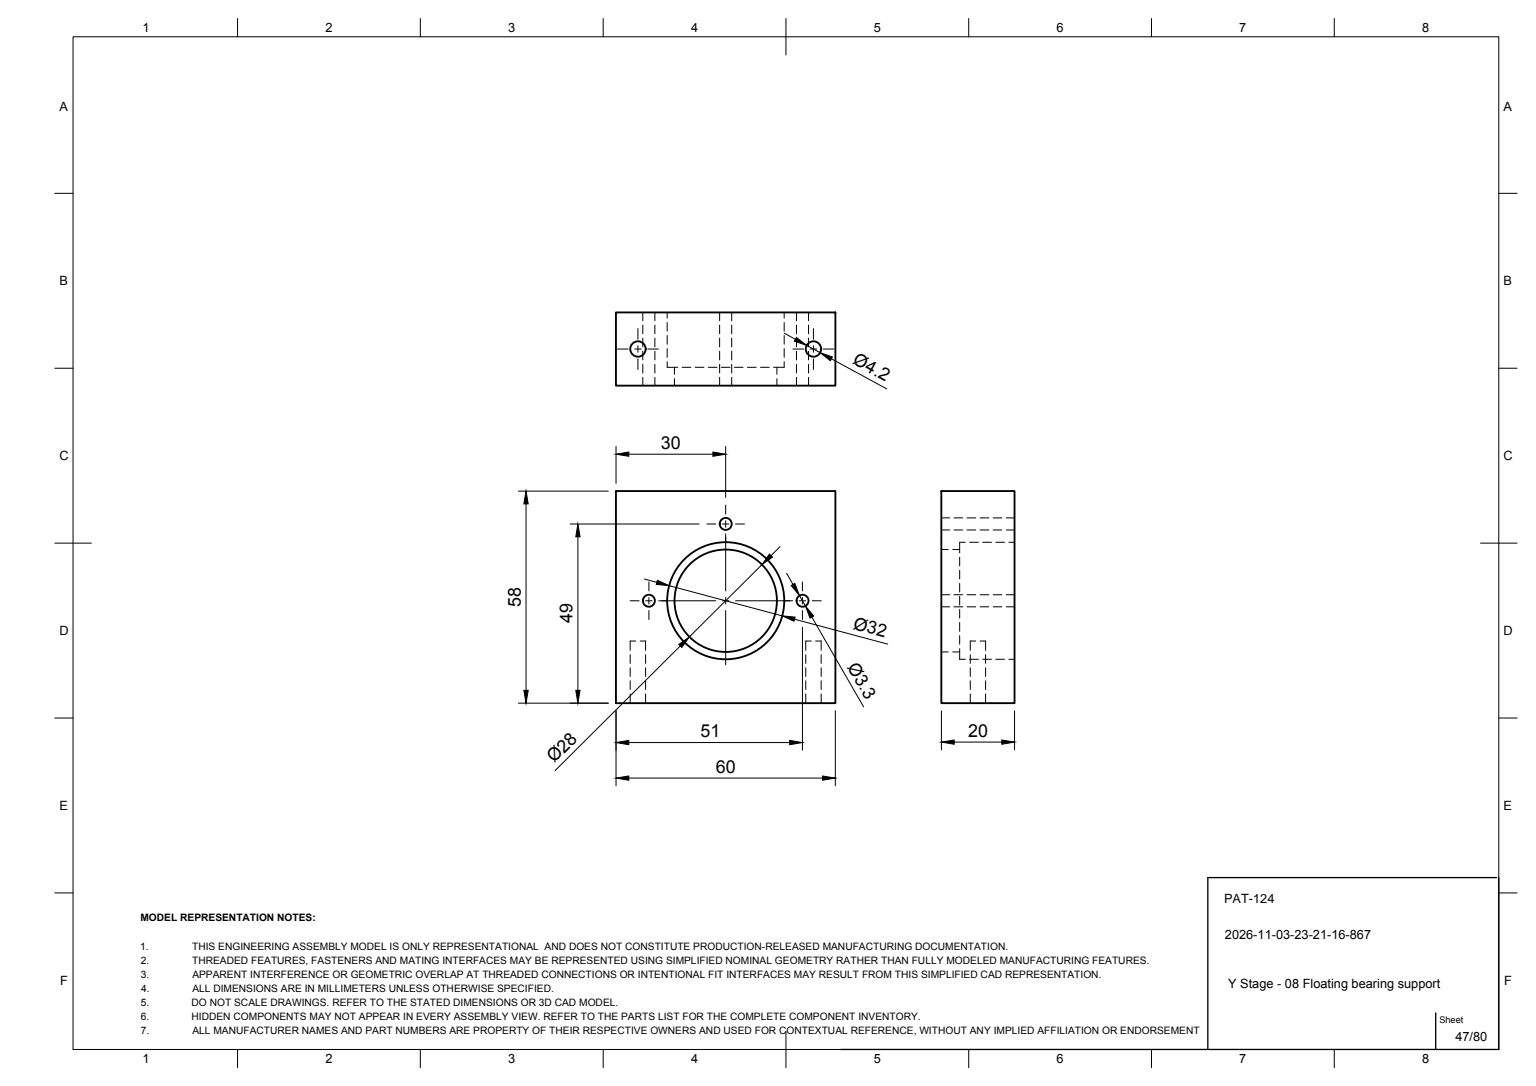
ISO-10303-21;
HEADER;
/* Generated by software containing ST-Developer
 * from STEP Tools, Inc. (www.steptools.com) 
 */

FILE_DESCRIPTION(
/* description */ ('XY cross-slide table'),
/* implementation_level */ '2;1');

FILE_NAME(
/* name */ 'Y Stage - 08 Floating bearing support.step',
/* time_stamp */ '2026-10-28T03:22:46-07:00',
/* author */ (''),
/* organization */ (''),
/* preprocessor_version */ 'ST-DEVELOPER v20.2',
/* originating_system */ 'Autodesk Translation Framework v15.17.0.0',
/* authorisation */ '');

FILE_SCHEMA (('AUTOMOTIVE_DESIGN { 1 0 10303 214 3 1 1 }'));
ENDSEC;

DATA;
#10=MECHANICAL_DESIGN_GEOMETRIC_PRESENTATION_REPRESENTATION('',(#1729),#62984);
#1548=SHAPE_REPRESENTATION_RELATIONSHIP('SRR','None',#63403,#1631);
#1631=ADVANCED_BREP_SHAPE_REPRESENTATION('',(#1838),#62940);
#1729=STYLED_ITEM('',(#63912),#1838);
#1838=MANIFOLD_SOLID_BREP('Body1',#23027);
#2143=FACE_BOUND('',#5155,.T.);
#2144=FACE_BOUND('',#5163,.T.);
#2145=FACE_BOUND('',#5164,.T.);
#2146=FACE_BOUND('',#5165,.T.);
#2147=FACE_BOUND('',#5166,.T.);
#2148=FACE_BOUND('',#5169,.T.);
#2149=FACE_BOUND('',#5170,.T.);
#2150=FACE_BOUND('',#5171,.T.);
#2151=FACE_BOUND('',#5172,.T.);
#2152=FACE_BOUND('',#5175,.T.);
#2153=FACE_BOUND('',#5176,.T.);
#2605=PLANE('',#25365);
#2606=PLANE('',#25372);
#2607=PLANE('',#25376);
#2608=PLANE('',#25377);
#2609=PLANE('',#25378);
#2610=PLANE('',#25379);
#2611=PLANE('',#25380);
#2612=PLANE('',#25381);
#2613=PLANE('',#25382);
#3580=FACE_OUTER_BOUND('',#5150,.T.);
#3581=FACE_OUTER_BOUND('',#5151,.T.);
#3582=FACE_OUTER_BOUND('',#5152,.T.);
#3583=FACE_OUTER_BOUND('',#5153,.T.);
#3584=FACE_OUTER_BOUND('',#5154,.T.);
#3585=FACE_OUTER_BOUND('',#5156,.T.);
#3586=FACE_OUTER_BOUND('',#5157,.T.);
#3587=FACE_OUTER_BOUND('',#5158,.T.);
#3588=FACE_OUTER_BOUND('',#5159,.T.);
#3589=FACE_OUTER_BOUND('',#5160,.T.);
#3590=FACE_OUTER_BOUND('',#5161,.T.);
#3591=FACE_OUTER_BOUND('',#5162,.T.);
#3592=FACE_OUTER_BOUND('',#5167,.T.);
#3593=FACE_OUTER_BOUND('',#5168,.T.);
#3594=FACE_OUTER_BOUND('',#5173,.T.);
#3595=FACE_OUTER_BOUND('',#5174,.T.);
#5150=EDGE_LOOP('',(#18226,#18227,#18228,#18229));
#5151=EDGE_LOOP('',(#18230,#18231,#18232,#18233));
#5152=EDGE_LOOP('',(#18234,#18235,#18236,#18237));
#5153=EDGE_LOOP('',(#18238,#18239,#18240,#18241));
#5154=EDGE_LOOP('',(#18242));
#5155=EDGE_LOOP('',(#18243));
#5156=EDGE_LOOP('',(#18244,#18245,#18246,#18247));
#5157=EDGE_LOOP('',(#18248,#18249,#18250,#18251));
#5158=EDGE_LOOP('',(#18252));
#5159=EDGE_LOOP('',(#18253,#18254,#18255,#18256));
#5160=EDGE_LOOP('',(#18257));
#5161=EDGE_LOOP('',(#18258,#18259,#18260,#18261));
#5162=EDGE_LOOP('',(#18262,#18263,#18264,#18265));
#5163=EDGE_LOOP('',(#18266));
#5164=EDGE_LOOP('',(#18267));
#5165=EDGE_LOOP('',(#18268));
#5166=EDGE_LOOP('',(#18269));
#5167=EDGE_LOOP('',(#18270,#18271,#18272,#18273));
#5168=EDGE_LOOP('',(#18274,#18275,#18276,#18277));
#5169=EDGE_LOOP('',(#18278));
#5170=EDGE_LOOP('',(#18279));
#5171=EDGE_LOOP('',(#18280));
#5172=EDGE_LOOP('',(#18281));
#5173=EDGE_LOOP('',(#18282,#18283,#18284,#18285));
#5174=EDGE_LOOP('',(#18286,#18287,#18288,#18289));
#5175=EDGE_LOOP('',(#18290));
#5176=EDGE_LOOP('',(#18291));
#6712=LINE('',#48100,#8199);
#6713=LINE('',#48106,#8200);
#6714=LINE('',#48112,#8201);
#6715=LINE('',#48118,#8202);
#6716=LINE('',#48125,#8203);
#6717=LINE('',#48131,#8204);
#6718=LINE('',#48138,#8205);
#6719=LINE('',#48144,#8206);
#6720=LINE('',#48146,#8207);
#6721=LINE('',#48148,#8208);
#6722=LINE('',#48149,#8209);
#6723=LINE('',#48152,#8210);
#6724=LINE('',#48154,#8211);
#6725=LINE('',#48155,#8212);
#6726=LINE('',#48158,#8213);
#6727=LINE('',#48160,#8214);
#6728=LINE('',#48161,#8215);
#6729=LINE('',#48163,#8216);
#6730=LINE('',#48164,#8217);
#8199=VECTOR('',#29977,0.165);
#8200=VECTOR('',#29984,0.165);
#8201=VECTOR('',#29991,0.165);
#8202=VECTOR('',#29998,1.6);
#8203=VECTOR('',#30007,1.4);
#8204=VECTOR('',#30014,0.21);
#8205=VECTOR('',#30023,0.21);
#8206=VECTOR('',#30030,1.);
#8207=VECTOR('',#30031,1.);
#8208=VECTOR('',#30032,1.);
#8209=VECTOR('',#30033,1.);
#8210=VECTOR('',#30036,1.);
#8211=VECTOR('',#30037,1.);
#8212=VECTOR('',#30038,1.);
#8213=VECTOR('',#30041,1.);
#8214=VECTOR('',#30042,1.);
#8215=VECTOR('',#30043,1.);
#8216=VECTOR('',#30046,1.);
#8217=VECTOR('',#30047,1.);
#9391=CIRCLE('',#25354,0.165);
#9392=CIRCLE('',#25355,0.165);
#9393=CIRCLE('',#25357,0.165);
#9394=CIRCLE('',#25358,0.165);
#9395=CIRCLE('',#25360,0.165);
#9396=CIRCLE('',#25361,0.165);
#9397=CIRCLE('',#25363,1.6);
#9398=CIRCLE('',#25364,1.6);
#9399=CIRCLE('',#25366,1.4);
#9400=CIRCLE('',#25368,1.4);
#9401=CIRCLE('',#25370,0.21);
#9402=CIRCLE('',#25371,0.21);
#9403=CIRCLE('',#25374,0.21);
#9404=CIRCLE('',#25375,0.21);
#10887=VERTEX_POINT('',#48097);
#10888=VERTEX_POINT('',#48099);
#10889=VERTEX_POINT('',#48103);
#10890=VERTEX_POINT('',#48105);
#10891=VERTEX_POINT('',#48109);
#10892=VERTEX_POINT('',#48111);
#10893=VERTEX_POINT('',#48115);
#10894=VERTEX_POINT('',#48117);
#10895=VERTEX_POINT('',#48121);
#10896=VERTEX_POINT('',#48124);
#10897=VERTEX_POINT('',#48128);
#10898=VERTEX_POINT('',#48130);
#10899=VERTEX_POINT('',#48135);
#10900=VERTEX_POINT('',#48137);
#10901=VERTEX_POINT('',#48142);
#10902=VERTEX_POINT('',#48143);
#10903=VERTEX_POINT('',#48145);
#10904=VERTEX_POINT('',#48147);
#10905=VERTEX_POINT('',#48151);
#10906=VERTEX_POINT('',#48153);
#10907=VERTEX_POINT('',#48157);
#10908=VERTEX_POINT('',#48159);
#13497=EDGE_CURVE('',#10887,#10887,#9391,.T.);
#13498=EDGE_CURVE('',#10887,#10888,#6712,.T.);
#13499=EDGE_CURVE('',#10888,#10888,#9392,.T.);
#13500=EDGE_CURVE('',#10889,#10889,#9393,.T.);
#13501=EDGE_CURVE('',#10889,#10890,#6713,.T.);
#13502=EDGE_CURVE('',#10890,#10890,#9394,.T.);
#13503=EDGE_CURVE('',#10891,#10891,#9395,.T.);
#13504=EDGE_CURVE('',#10891,#10892,#6714,.T.);
#13505=EDGE_CURVE('',#10892,#10892,#9396,.T.);
#13506=EDGE_CURVE('',#10893,#10893,#9397,.T.);
#13507=EDGE_CURVE('',#10893,#10894,#6715,.T.);
#13508=EDGE_CURVE('',#10894,#10894,#9398,.T.);
#13509=EDGE_CURVE('',#10895,#10895,#9399,.T.);
#13510=EDGE_CURVE('',#10895,#10896,#6716,.T.);
#13511=EDGE_CURVE('',#10896,#10896,#9400,.T.);
#13512=EDGE_CURVE('',#10897,#10897,#9401,.T.);
#13513=EDGE_CURVE('',#10897,#10898,#6717,.T.);
#13514=EDGE_CURVE('',#10898,#10898,#9402,.T.);
#13515=EDGE_CURVE('',#10899,#10899,#9403,.T.);
#13516=EDGE_CURVE('',#10899,#10900,#6718,.T.);
#13517=EDGE_CURVE('',#10900,#10900,#9404,.T.);
#13518=EDGE_CURVE('',#10901,#10902,#6719,.T.);
#13519=EDGE_CURVE('',#10902,#10903,#6720,.T.);
#13520=EDGE_CURVE('',#10904,#10903,#6721,.T.);
#13521=EDGE_CURVE('',#10901,#10904,#6722,.T.);
#13522=EDGE_CURVE('',#10905,#10901,#6723,.T.);
#13523=EDGE_CURVE('',#10906,#10904,#6724,.T.);
#13524=EDGE_CURVE('',#10905,#10906,#6725,.T.);
#13525=EDGE_CURVE('',#10907,#10905,#6726,.T.);
#13526=EDGE_CURVE('',#10908,#10906,#6727,.T.);
#13527=EDGE_CURVE('',#10907,#10908,#6728,.T.);
#13528=EDGE_CURVE('',#10902,#10907,#6729,.T.);
#13529=EDGE_CURVE('',#10903,#10908,#6730,.T.);
#18226=ORIENTED_EDGE('',*,*,#13497,.F.);
#18227=ORIENTED_EDGE('',*,*,#13498,.T.);
#18228=ORIENTED_EDGE('',*,*,#13499,.F.);
#18229=ORIENTED_EDGE('',*,*,#13498,.F.);
#18230=ORIENTED_EDGE('',*,*,#13500,.F.);
#18231=ORIENTED_EDGE('',*,*,#13501,.T.);
#18232=ORIENTED_EDGE('',*,*,#13502,.F.);
#18233=ORIENTED_EDGE('',*,*,#13501,.F.);
#18234=ORIENTED_EDGE('',*,*,#13503,.F.);
#18235=ORIENTED_EDGE('',*,*,#13504,.T.);
#18236=ORIENTED_EDGE('',*,*,#13505,.F.);
#18237=ORIENTED_EDGE('',*,*,#13504,.F.);
#18238=ORIENTED_EDGE('',*,*,#13506,.F.);
#18239=ORIENTED_EDGE('',*,*,#13507,.T.);
#18240=ORIENTED_EDGE('',*,*,#13508,.T.);
#18241=ORIENTED_EDGE('',*,*,#13507,.F.);
#18242=ORIENTED_EDGE('',*,*,#13508,.F.);
#18243=ORIENTED_EDGE('',*,*,#13509,.F.);
#18244=ORIENTED_EDGE('',*,*,#13509,.T.);
#18245=ORIENTED_EDGE('',*,*,#13510,.T.);
#18246=ORIENTED_EDGE('',*,*,#13511,.F.);
#18247=ORIENTED_EDGE('',*,*,#13510,.F.);
#18248=ORIENTED_EDGE('',*,*,#13512,.F.);
#18249=ORIENTED_EDGE('',*,*,#13513,.T.);
#18250=ORIENTED_EDGE('',*,*,#13514,.T.);
#18251=ORIENTED_EDGE('',*,*,#13513,.F.);
#18252=ORIENTED_EDGE('',*,*,#13514,.F.);
#18253=ORIENTED_EDGE('',*,*,#13515,.F.);
#18254=ORIENTED_EDGE('',*,*,#13516,.T.);
#18255=ORIENTED_EDGE('',*,*,#13517,.T.);
#18256=ORIENTED_EDGE('',*,*,#13516,.F.);
#18257=ORIENTED_EDGE('',*,*,#13517,.F.);
#18258=ORIENTED_EDGE('',*,*,#13518,.T.);
#18259=ORIENTED_EDGE('',*,*,#13519,.T.);
#18260=ORIENTED_EDGE('',*,*,#13520,.F.);
#18261=ORIENTED_EDGE('',*,*,#13521,.F.);
#18262=ORIENTED_EDGE('',*,*,#13522,.T.);
#18263=ORIENTED_EDGE('',*,*,#13521,.T.);
#18264=ORIENTED_EDGE('',*,*,#13523,.F.);
#18265=ORIENTED_EDGE('',*,*,#13524,.F.);
#18266=ORIENTED_EDGE('',*,*,#13499,.T.);
#18267=ORIENTED_EDGE('',*,*,#13502,.T.);
#18268=ORIENTED_EDGE('',*,*,#13505,.T.);
#18269=ORIENTED_EDGE('',*,*,#13511,.T.);
#18270=ORIENTED_EDGE('',*,*,#13525,.T.);
#18271=ORIENTED_EDGE('',*,*,#13524,.T.);
#18272=ORIENTED_EDGE('',*,*,#13526,.F.);
#18273=ORIENTED_EDGE('',*,*,#13527,.F.);
#18274=ORIENTED_EDGE('',*,*,#13528,.T.);
#18275=ORIENTED_EDGE('',*,*,#13527,.T.);
#18276=ORIENTED_EDGE('',*,*,#13529,.F.);
#18277=ORIENTED_EDGE('',*,*,#13519,.F.);
#18278=ORIENTED_EDGE('',*,*,#13497,.T.);
#18279=ORIENTED_EDGE('',*,*,#13500,.T.);
#18280=ORIENTED_EDGE('',*,*,#13503,.T.);
#18281=ORIENTED_EDGE('',*,*,#13506,.T.);
#18282=ORIENTED_EDGE('',*,*,#13529,.T.);
#18283=ORIENTED_EDGE('',*,*,#13526,.T.);
#18284=ORIENTED_EDGE('',*,*,#13523,.T.);
#18285=ORIENTED_EDGE('',*,*,#13520,.T.);
#18286=ORIENTED_EDGE('',*,*,#13528,.F.);
#18287=ORIENTED_EDGE('',*,*,#13518,.F.);
#18288=ORIENTED_EDGE('',*,*,#13522,.F.);
#18289=ORIENTED_EDGE('',*,*,#13525,.F.);
#18290=ORIENTED_EDGE('',*,*,#13512,.T.);
#18291=ORIENTED_EDGE('',*,*,#13515,.T.);
#21378=CYLINDRICAL_SURFACE('',#25353,0.165);
#21379=CYLINDRICAL_SURFACE('',#25356,0.165);
#21380=CYLINDRICAL_SURFACE('',#25359,0.165);
#21381=CYLINDRICAL_SURFACE('',#25362,1.6);
#21382=CYLINDRICAL_SURFACE('',#25367,1.4);
#21383=CYLINDRICAL_SURFACE('',#25369,0.21);
#21384=CYLINDRICAL_SURFACE('',#25373,0.21);
#22361=ADVANCED_FACE('',(#3580),#21378,.F.);
#22362=ADVANCED_FACE('',(#3581),#21379,.F.);
#22363=ADVANCED_FACE('',(#3582),#21380,.F.);
#22364=ADVANCED_FACE('',(#3583),#21381,.F.);
#22365=ADVANCED_FACE('',(#3584,#2143),#2605,.F.);
#22366=ADVANCED_FACE('',(#3585),#21382,.F.);
#22367=ADVANCED_FACE('',(#3586),#21383,.F.);
#22368=ADVANCED_FACE('',(#3587),#2606,.F.);
#22369=ADVANCED_FACE('',(#3588),#21384,.F.);
#22370=ADVANCED_FACE('',(#3589),#2607,.F.);
#22371=ADVANCED_FACE('',(#3590),#2608,.T.);
#22372=ADVANCED_FACE('',(#3591,#2144,#2145,#2146,#2147),#2609,.T.);
#22373=ADVANCED_FACE('',(#3592),#2610,.T.);
#22374=ADVANCED_FACE('',(#3593,#2148,#2149,#2150,#2151),#2611,.T.);
#22375=ADVANCED_FACE('',(#3594),#2612,.T.);
#22376=ADVANCED_FACE('',(#3595,#2152,#2153),#2613,.F.);
#23027=CLOSED_SHELL('',(#22361,#22362,#22363,#22364,#22365,#22366,#22367,
#22368,#22369,#22370,#22371,#22372,#22373,#22374,#22375,#22376));
#25352=AXIS2_PLACEMENT_3D('',#48095,#29971,#29972);
#25353=AXIS2_PLACEMENT_3D('',#48096,#29973,#29974);
#25354=AXIS2_PLACEMENT_3D('',#48098,#29975,#29976);
#25355=AXIS2_PLACEMENT_3D('',#48101,#29978,#29979);
#25356=AXIS2_PLACEMENT_3D('',#48102,#29980,#29981);
#25357=AXIS2_PLACEMENT_3D('',#48104,#29982,#29983);
#25358=AXIS2_PLACEMENT_3D('',#48107,#29985,#29986);
#25359=AXIS2_PLACEMENT_3D('',#48108,#29987,#29988);
#25360=AXIS2_PLACEMENT_3D('',#48110,#29989,#29990);
#25361=AXIS2_PLACEMENT_3D('',#48113,#29992,#29993);
#25362=AXIS2_PLACEMENT_3D('',#48114,#29994,#29995);
#25363=AXIS2_PLACEMENT_3D('',#48116,#29996,#29997);
#25364=AXIS2_PLACEMENT_3D('',#48119,#29999,#30000);
#25365=AXIS2_PLACEMENT_3D('',#48120,#30001,#30002);
#25366=AXIS2_PLACEMENT_3D('',#48122,#30003,#30004);
#25367=AXIS2_PLACEMENT_3D('',#48123,#30005,#30006);
#25368=AXIS2_PLACEMENT_3D('',#48126,#30008,#30009);
#25369=AXIS2_PLACEMENT_3D('',#48127,#30010,#30011);
#25370=AXIS2_PLACEMENT_3D('',#48129,#30012,#30013);
#25371=AXIS2_PLACEMENT_3D('',#48132,#30015,#30016);
#25372=AXIS2_PLACEMENT_3D('',#48133,#30017,#30018);
#25373=AXIS2_PLACEMENT_3D('',#48134,#30019,#30020);
#25374=AXIS2_PLACEMENT_3D('',#48136,#30021,#30022);
#25375=AXIS2_PLACEMENT_3D('',#48139,#30024,#30025);
#25376=AXIS2_PLACEMENT_3D('',#48140,#30026,#30027);
#25377=AXIS2_PLACEMENT_3D('',#48141,#30028,#30029);
#25378=AXIS2_PLACEMENT_3D('',#48150,#30034,#30035);
#25379=AXIS2_PLACEMENT_3D('',#48156,#30039,#30040);
#25380=AXIS2_PLACEMENT_3D('',#48162,#30044,#30045);
#25381=AXIS2_PLACEMENT_3D('',#48165,#30048,#30049);
#25382=AXIS2_PLACEMENT_3D('',#48166,#30050,#30051);
#29971=DIRECTION('axis',(0.,0.,1.));
#29972=DIRECTION('refdir',(1.,0.,0.));
#29973=DIRECTION('center_axis',(1.,0.,0.));
#29974=DIRECTION('ref_axis',(0.,0.,-1.));
#29975=DIRECTION('center_axis',(1.,0.,0.));
#29976=DIRECTION('ref_axis',(0.,0.,-1.));
#29977=DIRECTION('',(1.,0.,0.));
#29978=DIRECTION('center_axis',(-1.,0.,0.));
#29979=DIRECTION('ref_axis',(0.,0.,-1.));
#29980=DIRECTION('center_axis',(1.,0.,0.));
#29981=DIRECTION('ref_axis',(0.,0.,-1.));
#29982=DIRECTION('center_axis',(1.,0.,0.));
#29983=DIRECTION('ref_axis',(0.,0.,-1.));
#29984=DIRECTION('',(1.,0.,0.));
#29985=DIRECTION('center_axis',(-1.,0.,0.));
#29986=DIRECTION('ref_axis',(0.,0.,-1.));
#29987=DIRECTION('center_axis',(1.,0.,0.));
#29988=DIRECTION('ref_axis',(0.,0.,-1.));
#29989=DIRECTION('center_axis',(1.,0.,0.));
#29990=DIRECTION('ref_axis',(0.,0.,-1.));
#29991=DIRECTION('',(1.,0.,0.));
#29992=DIRECTION('center_axis',(-1.,0.,0.));
#29993=DIRECTION('ref_axis',(0.,0.,-1.));
#29994=DIRECTION('center_axis',(1.,0.,0.));
#29995=DIRECTION('ref_axis',(0.,0.,-1.));
#29996=DIRECTION('center_axis',(1.,0.,0.));
#29997=DIRECTION('ref_axis',(0.,0.,-1.));
#29998=DIRECTION('',(1.,0.,0.));
#29999=DIRECTION('center_axis',(1.,0.,0.));
#30000=DIRECTION('ref_axis',(0.,0.,-1.));
#30001=DIRECTION('center_axis',(1.,0.,0.));
#30002=DIRECTION('ref_axis',(0.,0.,-1.));
#30003=DIRECTION('center_axis',(-1.,0.,0.));
#30004=DIRECTION('ref_axis',(0.,0.,-1.));
#30005=DIRECTION('center_axis',(1.,0.,0.));
#30006=DIRECTION('ref_axis',(0.,0.,-1.));
#30007=DIRECTION('',(1.,0.,0.));
#30008=DIRECTION('center_axis',(-1.,0.,0.));
#30009=DIRECTION('ref_axis',(0.,0.,-1.));
#30010=DIRECTION('center_axis',(0.,0.,1.));
#30011=DIRECTION('ref_axis',(1.,0.,0.));
#30012=DIRECTION('center_axis',(0.,0.,1.));
#30013=DIRECTION('ref_axis',(1.,0.,0.));
#30014=DIRECTION('',(0.,0.,1.));
#30015=DIRECTION('center_axis',(0.,0.,1.));
#30016=DIRECTION('ref_axis',(1.,0.,0.));
#30017=DIRECTION('center_axis',(0.,0.,1.));
#30018=DIRECTION('ref_axis',(1.,0.,0.));
#30019=DIRECTION('center_axis',(0.,0.,1.));
#30020=DIRECTION('ref_axis',(1.,0.,0.));
#30021=DIRECTION('center_axis',(0.,0.,1.));
#30022=DIRECTION('ref_axis',(1.,0.,0.));
#30023=DIRECTION('',(0.,0.,1.));
#30024=DIRECTION('center_axis',(0.,0.,1.));
#30025=DIRECTION('ref_axis',(1.,0.,0.));
#30026=DIRECTION('center_axis',(0.,0.,1.));
#30027=DIRECTION('ref_axis',(1.,0.,0.));
#30028=DIRECTION('center_axis',(0.,1.,0.));
#30029=DIRECTION('ref_axis',(-1.,0.,0.));
#30030=DIRECTION('',(-1.,0.,0.));
#30031=DIRECTION('',(0.,0.,1.));
#30032=DIRECTION('',(-1.,0.,0.));
#30033=DIRECTION('',(0.,0.,1.));
#30034=DIRECTION('center_axis',(1.,0.,0.));
#30035=DIRECTION('ref_axis',(0.,1.,0.));
#30036=DIRECTION('',(0.,1.,0.));
#30037=DIRECTION('',(0.,1.,0.));
#30038=DIRECTION('',(0.,0.,1.));
#30039=DIRECTION('center_axis',(0.,-1.,0.));
#30040=DIRECTION('ref_axis',(1.,0.,0.));
#30041=DIRECTION('',(1.,0.,0.));
#30042=DIRECTION('',(1.,0.,0.));
#30043=DIRECTION('',(0.,0.,1.));
#30044=DIRECTION('center_axis',(-1.,0.,0.));
#30045=DIRECTION('ref_axis',(0.,-1.,0.));
#30046=DIRECTION('',(0.,-1.,0.));
#30047=DIRECTION('',(0.,-1.,0.));
#30048=DIRECTION('center_axis',(0.,0.,1.));
#30049=DIRECTION('ref_axis',(1.,0.,0.));
#30050=DIRECTION('center_axis',(0.,0.,1.));
#30051=DIRECTION('ref_axis',(1.,0.,0.));
#48095=CARTESIAN_POINT('',(0.,0.,0.));
#48096=CARTESIAN_POINT('Origin',(1.9,-2.1,4.));
#48097=CARTESIAN_POINT('',(2.,-2.1,4.165));
#48098=CARTESIAN_POINT('Origin',(2.,-2.1,4.));
#48099=CARTESIAN_POINT('',(4.,-2.1,4.165));
#48100=CARTESIAN_POINT('',(1.9,-2.1,4.165));
#48101=CARTESIAN_POINT('Origin',(4.,-2.1,4.));
#48102=CARTESIAN_POINT('Origin',(1.9,2.1,4.));
#48103=CARTESIAN_POINT('',(2.,2.1,4.165));
#48104=CARTESIAN_POINT('Origin',(2.,2.1,4.));
#48105=CARTESIAN_POINT('',(4.,2.1,4.165));
#48106=CARTESIAN_POINT('',(1.9,2.1,4.165));
#48107=CARTESIAN_POINT('Origin',(4.,2.1,4.));
#48108=CARTESIAN_POINT('Origin',(1.9,0.,6.1));
#48109=CARTESIAN_POINT('',(2.,-2.02066721859313E-17,6.265));
#48110=CARTESIAN_POINT('Origin',(2.,0.,6.1));
#48111=CARTESIAN_POINT('',(4.,2.02066721859313E-17,6.265));
#48112=CARTESIAN_POINT('',(1.9,-2.02066721859313E-17,6.265));
#48113=CARTESIAN_POINT('Origin',(4.,0.,6.1));
#48114=CARTESIAN_POINT('Origin',(1.9,0.,4.));
#48115=CARTESIAN_POINT('',(2.,-1.95943487863577E-16,5.6));
#48116=CARTESIAN_POINT('Origin',(2.,0.,4.));
#48117=CARTESIAN_POINT('',(3.5,-1.95943487863577E-16,5.6));
#48118=CARTESIAN_POINT('',(1.9,-1.95943487863577E-16,5.6));
#48119=CARTESIAN_POINT('Origin',(3.5,0.,4.));
#48120=CARTESIAN_POINT('Origin',(3.5,0.,4.));
#48121=CARTESIAN_POINT('',(3.5,1.71450551880629E-16,5.4));
#48122=CARTESIAN_POINT('Origin',(3.5,0.,4.));
#48123=CARTESIAN_POINT('Origin',(1.9,0.,4.));
#48124=CARTESIAN_POINT('',(4.,1.71450551880629E-16,5.4));
#48125=CARTESIAN_POINT('',(1.9,-1.71450551880629E-16,5.4));
#48126=CARTESIAN_POINT('Origin',(4.,0.,4.));
#48127=CARTESIAN_POINT('Origin',(3.,-2.4,1.1));
#48128=CARTESIAN_POINT('',(2.79,-2.4,1.2));
#48129=CARTESIAN_POINT('Origin',(3.,-2.4,1.2));
#48130=CARTESIAN_POINT('',(2.79,-2.4,2.9));
#48131=CARTESIAN_POINT('',(2.79,-2.4,1.1));
#48132=CARTESIAN_POINT('Origin',(3.,-2.4,2.9));
#48133=CARTESIAN_POINT('Origin',(3.,-2.4,2.9));
#48134=CARTESIAN_POINT('Origin',(3.,2.4,1.1));
#48135=CARTESIAN_POINT('',(2.79,2.4,1.2));
#48136=CARTESIAN_POINT('Origin',(3.,2.4,1.2));
#48137=CARTESIAN_POINT('',(2.79,2.4,2.9));
#48138=CARTESIAN_POINT('',(2.79,2.4,1.1));
#48139=CARTESIAN_POINT('Origin',(3.,2.4,2.9));
#48140=CARTESIAN_POINT('Origin',(3.,2.4,2.9));
#48141=CARTESIAN_POINT('Origin',(4.,3.,1.2));
#48142=CARTESIAN_POINT('',(4.,3.,1.2));
#48143=CARTESIAN_POINT('',(2.,3.,1.2));
#48144=CARTESIAN_POINT('',(4.,3.,1.2));
#48145=CARTESIAN_POINT('',(2.,3.,7.));
#48146=CARTESIAN_POINT('',(2.,3.,1.2));
#48147=CARTESIAN_POINT('',(4.,3.,7.));
#48148=CARTESIAN_POINT('',(4.,3.,7.));
#48149=CARTESIAN_POINT('',(4.,3.,1.2));
#48150=CARTESIAN_POINT('Origin',(4.,-3.,1.2));
#48151=CARTESIAN_POINT('',(4.,-3.,1.2));
#48152=CARTESIAN_POINT('',(4.,-3.,1.2));
#48153=CARTESIAN_POINT('',(4.,-3.,7.));
#48154=CARTESIAN_POINT('',(4.,-3.,7.));
#48155=CARTESIAN_POINT('',(4.,-3.,1.2));
#48156=CARTESIAN_POINT('Origin',(2.,-3.,1.2));
#48157=CARTESIAN_POINT('',(2.,-3.,1.2));
#48158=CARTESIAN_POINT('',(2.,-3.,1.2));
#48159=CARTESIAN_POINT('',(2.,-3.,7.));
#48160=CARTESIAN_POINT('',(2.,-3.,7.));
#48161=CARTESIAN_POINT('',(2.,-3.,1.2));
#48162=CARTESIAN_POINT('Origin',(2.,3.,1.2));
#48163=CARTESIAN_POINT('',(2.,3.,1.2));
#48164=CARTESIAN_POINT('',(2.,3.,7.));
#48165=CARTESIAN_POINT('Origin',(3.,0.,7.));
#48166=CARTESIAN_POINT('Origin',(3.,0.,1.2));
#62841=UNCERTAINTY_MEASURE_WITH_UNIT(LENGTH_MEASURE(0.001),#62985,
'DISTANCE_ACCURACY_VALUE',
'Maximum model space distance between geometric entities at asserted c
onnectivities');
#62885=UNCERTAINTY_MEASURE_WITH_UNIT(LENGTH_MEASURE(0.001),#62985,
'DISTANCE_ACCURACY_VALUE',
'Maximum model space distance between geometric entities at asserted c
onnectivities');
#62940=(
GEOMETRIC_REPRESENTATION_CONTEXT(3)
GLOBAL_UNCERTAINTY_ASSIGNED_CONTEXT((#62841))
GLOBAL_UNIT_ASSIGNED_CONTEXT((#62985,#62987,#62988))
REPRESENTATION_CONTEXT('','3D')
);
#62984=(
GEOMETRIC_REPRESENTATION_CONTEXT(3)
GLOBAL_UNCERTAINTY_ASSIGNED_CONTEXT((#62885))
GLOBAL_UNIT_ASSIGNED_CONTEXT((#62985,#62987,#62988))
REPRESENTATION_CONTEXT('','3D')
);
#62985=(
LENGTH_UNIT()
NAMED_UNIT(*)
SI_UNIT(.CENTI.,.METRE.)
);
#62987=(
NAMED_UNIT(*)
PLANE_ANGLE_UNIT()
SI_UNIT($,.RADIAN.)
);
#62988=(
NAMED_UNIT(*)
SI_UNIT($,.STERADIAN.)
SOLID_ANGLE_UNIT()
);
#63043=SHAPE_DEFINITION_REPRESENTATION(#63221,#63403);
#63221=PRODUCT_DEFINITION_SHAPE('',$,#63502);
#63403=SHAPE_REPRESENTATION('',(#25352),#62940);
#63447=PRODUCT_DEFINITION_CONTEXT('part definition',#63743,'design');
#63502=PRODUCT_DEFINITION('Y Stage - 08 Floating bearing support',
'Y Stage - 08 Floating bearing support',#63600,#63447);
#63600=PRODUCT_DEFINITION_FORMATION('',$,#63799);
#63743=APPLICATION_CONTEXT(
'Core Data for Automotive Mechanical Design Process');
#63744=PRODUCT_CONTEXT('part definition',#63743,'mechanical');
#63799=PRODUCT('Y Stage - 08 Floating bearing support',
'Y Stage - 08 Floating bearing support',
'Y Stage - 08 Floating bearing support',(#63744));
#63906=COLOUR_RGB('Grey',0.48,0.52,0.57);
#63907=FILL_AREA_STYLE_COLOUR('',#63906);
#63908=FILL_AREA_STYLE('',(#63907));
#63909=SURFACE_STYLE_FILL_AREA(#63908);
#63910=SURFACE_SIDE_STYLE('',(#63909));
#63911=SURFACE_STYLE_USAGE(.BOTH.,#63910);
#63912=PRESENTATION_STYLE_ASSIGNMENT((#63911));
ENDSEC;
END-ISO-10303-21;
